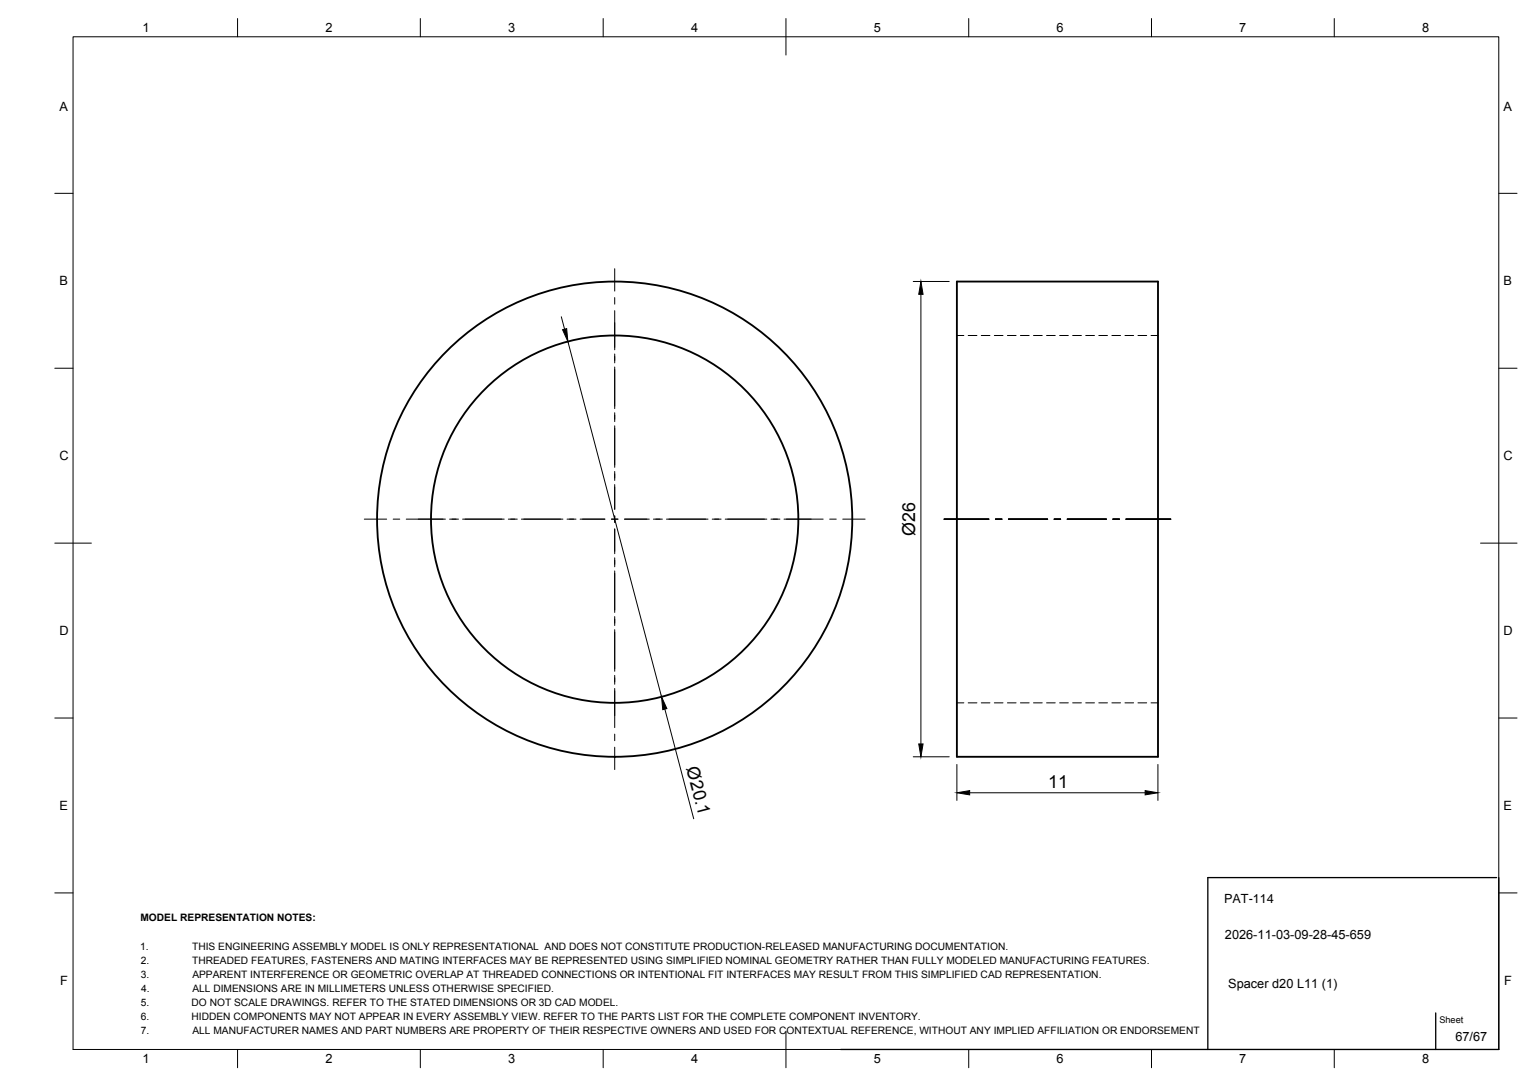
ISO-10303-21;
HEADER;
/* Generated by software containing ST-Developer
 * from STEP Tools, Inc. (www.steptools.com) 
 */

FILE_DESCRIPTION(
/* description */ ('Two-stage gear reducer in split housing'),
/* implementation_level */ '2;1');

FILE_NAME(
/* name */ 'Spacer d20 L11 (1).step',
/* time_stamp */ '2026-10-28T03:22:31-07:00',
/* author */ (''),
/* organization */ (''),
/* preprocessor_version */ 'ST-DEVELOPER v20.2',
/* originating_system */ 'Autodesk Translation Framework v15.17.0.0',
/* authorisation */ '');

FILE_SCHEMA (('AUTOMOTIVE_DESIGN { 1 0 10303 214 3 1 1 }'));
ENDSEC;

DATA;
#10=MECHANICAL_DESIGN_GEOMETRIC_PRESENTATION_REPRESENTATION('',(#1301),#73366);
#1174=SHAPE_REPRESENTATION_RELATIONSHIP('SRR','None',#73666,#1230);
#1230=ADVANCED_BREP_SHAPE_REPRESENTATION('',(#1370),#73362);
#1301=STYLED_ITEM('',(#73974),#1370);
#1370=MANIFOLD_SOLID_BREP('Body1',#16191);
#1596=FACE_BOUND('',#3859,.T.);
#1597=FACE_BOUND('',#3861,.T.);
#1935=PLANE('',#18215);
#1936=PLANE('',#18216);
#2721=FACE_OUTER_BOUND('',#3856,.T.);
#2722=FACE_OUTER_BOUND('',#3857,.T.);
#2723=FACE_OUTER_BOUND('',#3858,.T.);
#2724=FACE_OUTER_BOUND('',#3860,.T.);
#3856=EDGE_LOOP('',(#13807,#13808,#13809,#13810));
#3857=EDGE_LOOP('',(#13811,#13812,#13813,#13814));
#3858=EDGE_LOOP('',(#13815));
#3859=EDGE_LOOP('',(#13816));
#3860=EDGE_LOOP('',(#13817));
#3861=EDGE_LOOP('',(#13818));
#4862=LINE('',#49530,#5886);
#4863=LINE('',#49536,#5887);
#5886=VECTOR('',#22062,1.005);
#5887=VECTOR('',#22069,1.3);
#6732=CIRCLE('',#18210,1.005);
#6733=CIRCLE('',#18211,1.005);
#6734=CIRCLE('',#18213,1.3);
#6735=CIRCLE('',#18214,1.3);
#7941=VERTEX_POINT('',#49527);
#7942=VERTEX_POINT('',#49529);
#7943=VERTEX_POINT('',#49533);
#7944=VERTEX_POINT('',#49535);
#9957=EDGE_CURVE('',#7941,#7941,#6732,.T.);
#9958=EDGE_CURVE('',#7941,#7942,#4862,.T.);
#9959=EDGE_CURVE('',#7942,#7942,#6733,.T.);
#9960=EDGE_CURVE('',#7943,#7943,#6734,.T.);
#9961=EDGE_CURVE('',#7943,#7944,#4863,.T.);
#9962=EDGE_CURVE('',#7944,#7944,#6735,.T.);
#13807=ORIENTED_EDGE('',*,*,#9957,.F.);
#13808=ORIENTED_EDGE('',*,*,#9958,.T.);
#13809=ORIENTED_EDGE('',*,*,#9959,.T.);
#13810=ORIENTED_EDGE('',*,*,#9958,.F.);
#13811=ORIENTED_EDGE('',*,*,#9960,.F.);
#13812=ORIENTED_EDGE('',*,*,#9961,.T.);
#13813=ORIENTED_EDGE('',*,*,#9962,.T.);
#13814=ORIENTED_EDGE('',*,*,#9961,.F.);
#13815=ORIENTED_EDGE('',*,*,#9960,.T.);
#13816=ORIENTED_EDGE('',*,*,#9957,.T.);
#13817=ORIENTED_EDGE('',*,*,#9962,.F.);
#13818=ORIENTED_EDGE('',*,*,#9959,.F.);
#15164=CYLINDRICAL_SURFACE('',#18209,1.005);
#15165=CYLINDRICAL_SURFACE('',#18212,1.3);
#15928=ADVANCED_FACE('',(#2721),#15164,.F.);
#15929=ADVANCED_FACE('',(#2722),#15165,.T.);
#15930=ADVANCED_FACE('',(#2723,#1596),#1935,.T.);
#15931=ADVANCED_FACE('',(#2724,#1597),#1936,.F.);
#16191=CLOSED_SHELL('',(#15928,#15929,#15930,#15931));
#18208=AXIS2_PLACEMENT_3D('',#49525,#22056,#22057);
#18209=AXIS2_PLACEMENT_3D('',#49526,#22058,#22059);
#18210=AXIS2_PLACEMENT_3D('',#49528,#22060,#22061);
#18211=AXIS2_PLACEMENT_3D('',#49531,#22063,#22064);
#18212=AXIS2_PLACEMENT_3D('',#49532,#22065,#22066);
#18213=AXIS2_PLACEMENT_3D('',#49534,#22067,#22068);
#18214=AXIS2_PLACEMENT_3D('',#49537,#22070,#22071);
#18215=AXIS2_PLACEMENT_3D('',#49538,#22072,#22073);
#18216=AXIS2_PLACEMENT_3D('',#49539,#22074,#22075);
#22056=DIRECTION('axis',(0.,0.,1.));
#22057=DIRECTION('refdir',(1.,0.,0.));
#22058=DIRECTION('center_axis',(0.,1.,0.));
#22059=DIRECTION('ref_axis',(1.,0.,0.));
#22060=DIRECTION('center_axis',(0.,-1.,0.));
#22061=DIRECTION('ref_axis',(1.,0.,0.));
#22062=DIRECTION('',(0.,-1.,0.));
#22063=DIRECTION('center_axis',(0.,-1.,0.));
#22064=DIRECTION('ref_axis',(1.,0.,0.));
#22065=DIRECTION('center_axis',(0.,1.,0.));
#22066=DIRECTION('ref_axis',(1.,0.,0.));
#22067=DIRECTION('center_axis',(0.,1.,0.));
#22068=DIRECTION('ref_axis',(1.,0.,0.));
#22069=DIRECTION('',(0.,-1.,0.));
#22070=DIRECTION('center_axis',(0.,1.,0.));
#22071=DIRECTION('ref_axis',(1.,0.,0.));
#22072=DIRECTION('center_axis',(0.,1.,0.));
#22073=DIRECTION('ref_axis',(1.,0.,0.));
#22074=DIRECTION('center_axis',(0.,1.,0.));
#22075=DIRECTION('ref_axis',(1.,0.,0.));
#49525=CARTESIAN_POINT('',(0.,0.,0.));
#49526=CARTESIAN_POINT('Origin',(12.,4.2,10.));
#49527=CARTESIAN_POINT('',(10.995,5.3,10.));
#49528=CARTESIAN_POINT('Origin',(12.,5.3,10.));
#49529=CARTESIAN_POINT('',(10.995,4.2,10.));
#49530=CARTESIAN_POINT('',(10.995,4.2,10.));
#49531=CARTESIAN_POINT('Origin',(12.,4.2,10.));
#49532=CARTESIAN_POINT('Origin',(12.,4.2,10.));
#49533=CARTESIAN_POINT('',(10.7,5.3,10.));
#49534=CARTESIAN_POINT('Origin',(12.,5.3,10.));
#49535=CARTESIAN_POINT('',(10.7,4.2,10.));
#49536=CARTESIAN_POINT('',(10.7,4.2,10.));
#49537=CARTESIAN_POINT('Origin',(12.,4.2,10.));
#49538=CARTESIAN_POINT('Origin',(12.,5.3,10.));
#49539=CARTESIAN_POINT('Origin',(12.,4.2,10.));
#73298=UNCERTAINTY_MEASURE_WITH_UNIT(LENGTH_MEASURE(0.001),#73367,
'DISTANCE_ACCURACY_VALUE',
'Maximum model space distance between geometric entities at asserted c
onnectivities');
#73302=UNCERTAINTY_MEASURE_WITH_UNIT(LENGTH_MEASURE(0.001),#73367,
'DISTANCE_ACCURACY_VALUE',
'Maximum model space distance between geometric entities at asserted c
onnectivities');
#73362=(
GEOMETRIC_REPRESENTATION_CONTEXT(3)
GLOBAL_UNCERTAINTY_ASSIGNED_CONTEXT((#73298))
GLOBAL_UNIT_ASSIGNED_CONTEXT((#73367,#73369,#73370))
REPRESENTATION_CONTEXT('','3D')
);
#73366=(
GEOMETRIC_REPRESENTATION_CONTEXT(3)
GLOBAL_UNCERTAINTY_ASSIGNED_CONTEXT((#73302))
GLOBAL_UNIT_ASSIGNED_CONTEXT((#73367,#73369,#73370))
REPRESENTATION_CONTEXT('','3D')
);
#73367=(
LENGTH_UNIT()
NAMED_UNIT(*)
SI_UNIT(.CENTI.,.METRE.)
);
#73369=(
NAMED_UNIT(*)
PLANE_ANGLE_UNIT()
SI_UNIT($,.RADIAN.)
);
#73370=(
NAMED_UNIT(*)
SI_UNIT($,.STERADIAN.)
SOLID_ANGLE_UNIT()
);
#73430=SHAPE_DEFINITION_REPRESENTATION(#73563,#73666);
#73563=PRODUCT_DEFINITION_SHAPE('',$,#73730);
#73666=SHAPE_REPRESENTATION('',(#18208),#73362);
#73670=PRODUCT_DEFINITION_CONTEXT('part definition',#73861,'design');
#73730=PRODUCT_DEFINITION('Spacer d20 L11 (1)','Spacer d20 L11 (1)',#73793,
#73670);
#73793=PRODUCT_DEFINITION_FORMATION('',$,#73922);
#73861=APPLICATION_CONTEXT(
'Core Data for Automotive Mechanical Design Process');
#73862=PRODUCT_CONTEXT('part definition',#73861,'mechanical');
#73922=PRODUCT('Spacer d20 L11 (1)','Spacer d20 L11 (1)','Spacer d20 L11 (1)',
(#73862));
#73968=COLOUR_RGB('Light Blue',0.38,0.62,0.78);
#73969=FILL_AREA_STYLE_COLOUR('',#73968);
#73970=FILL_AREA_STYLE('',(#73969));
#73971=SURFACE_STYLE_FILL_AREA(#73970);
#73972=SURFACE_SIDE_STYLE('',(#73971));
#73973=SURFACE_STYLE_USAGE(.BOTH.,#73972);
#73974=PRESENTATION_STYLE_ASSIGNMENT((#73973));
ENDSEC;
END-ISO-10303-21;
